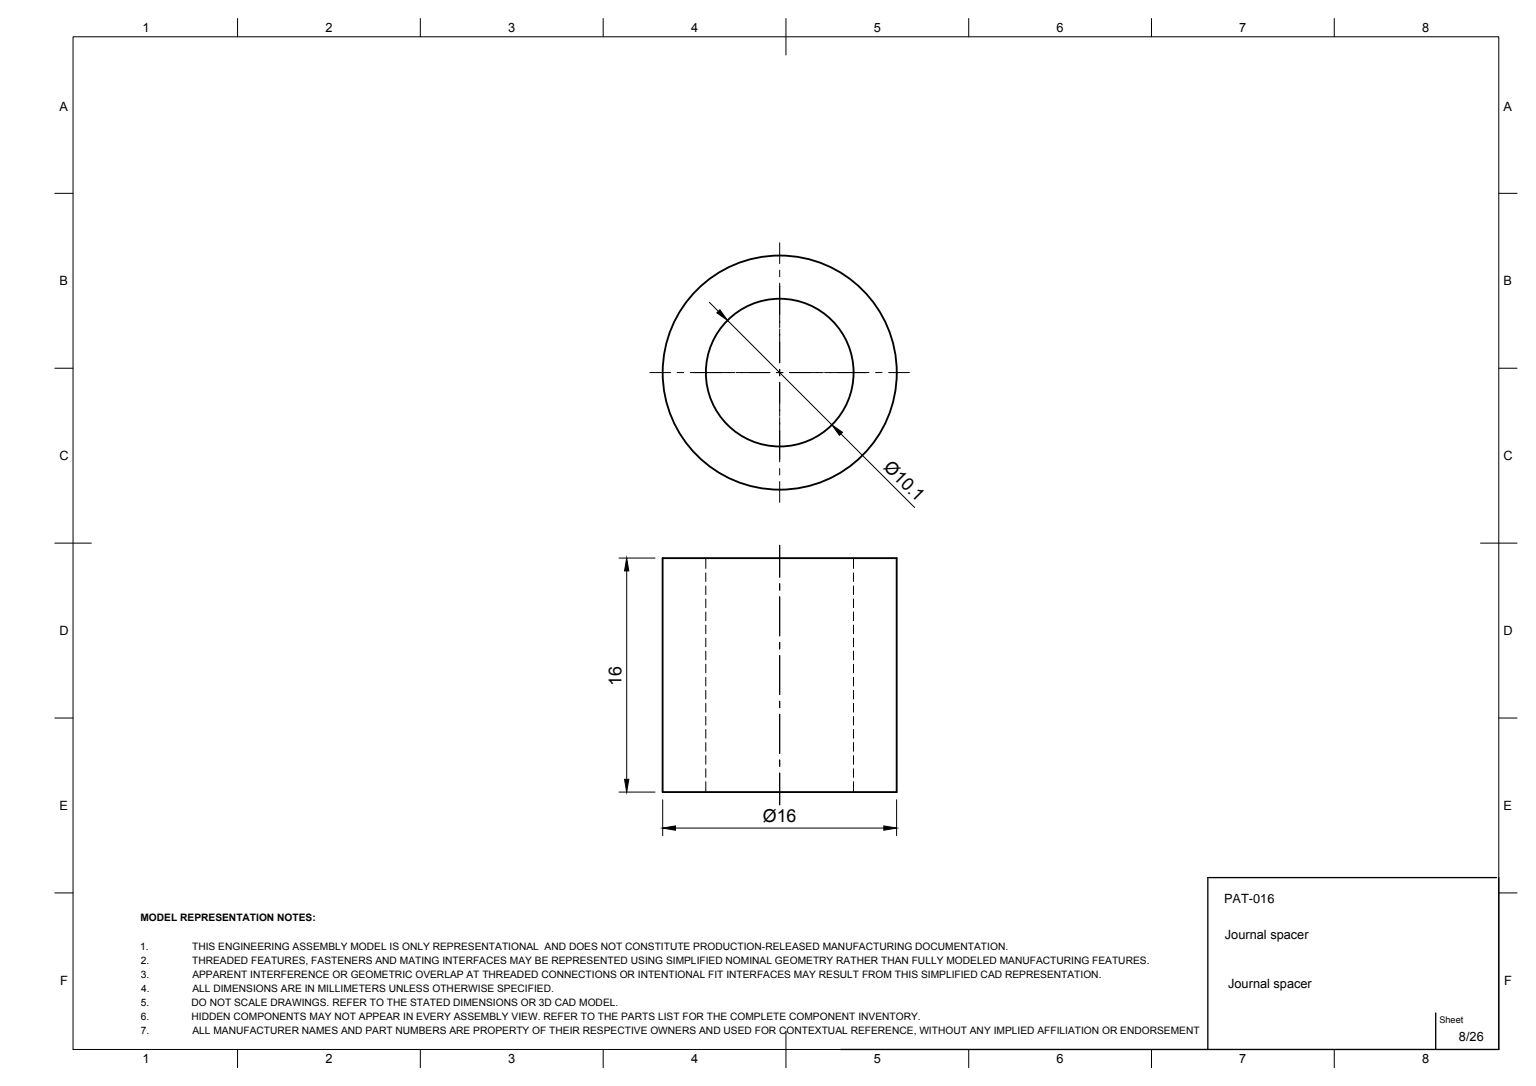
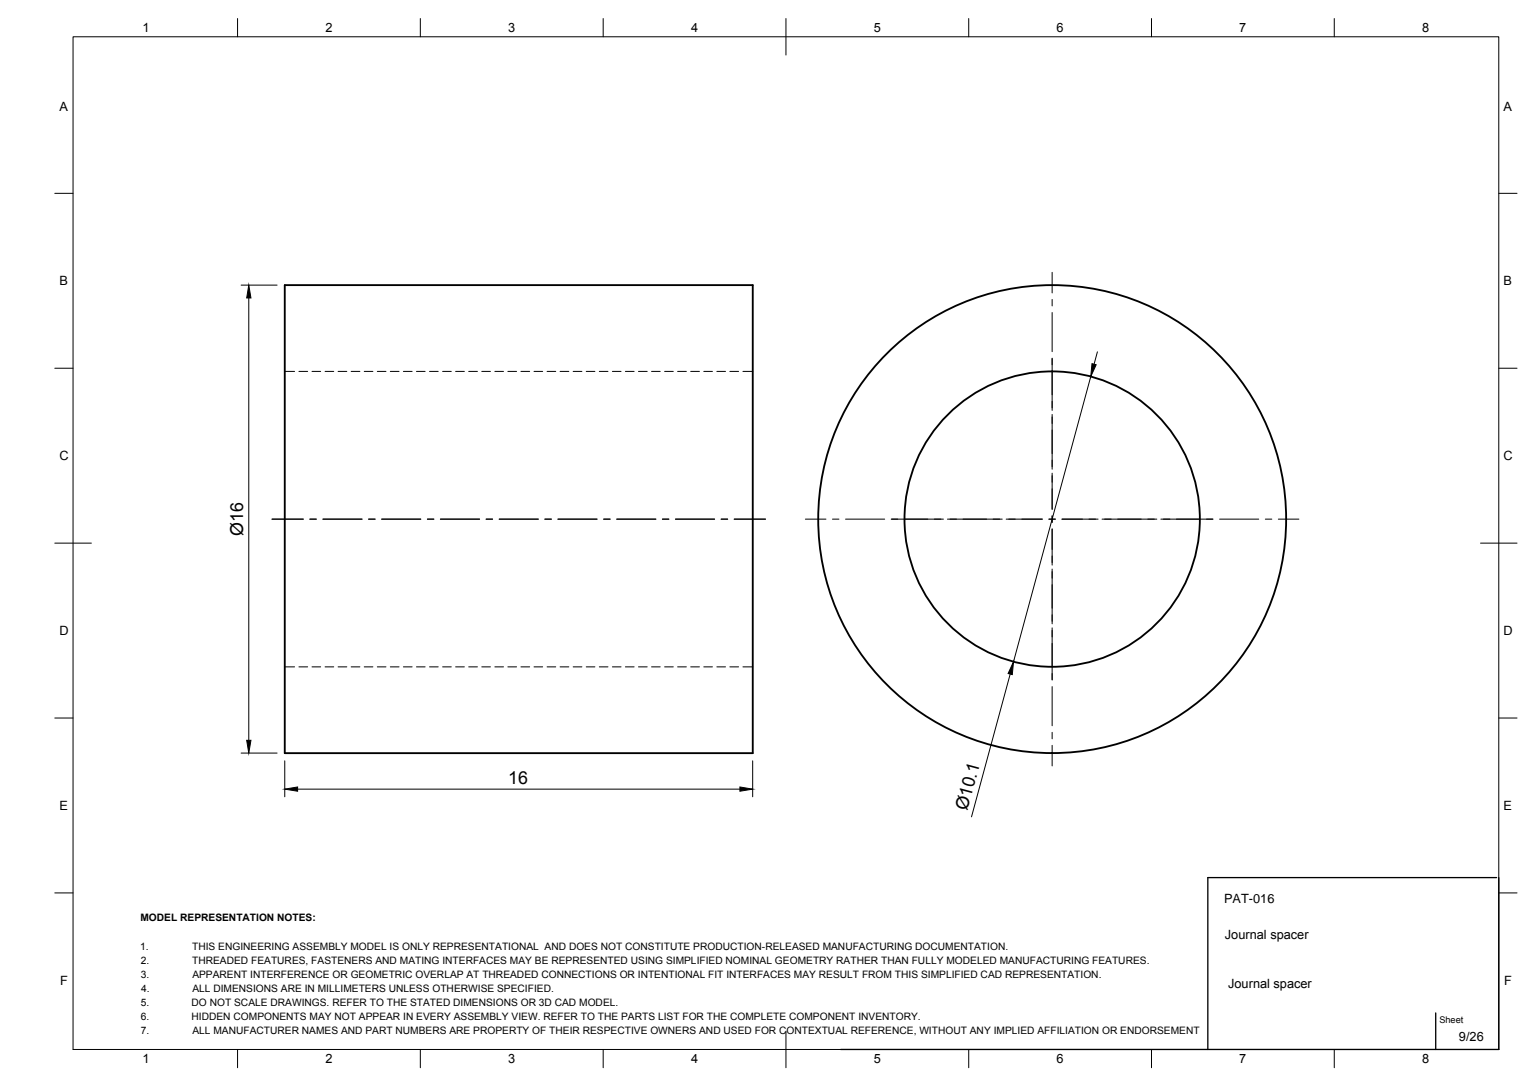
ISO-10303-21;
HEADER;
/* Generated by software containing ST-Developer
 * from STEP Tools, Inc. (www.steptools.com) 
 */

FILE_DESCRIPTION(
/* description */ ('Bracket-mounted idler roller'),
/* implementation_level */ '2;1');

FILE_NAME(
/* name */ 'Journal spacer.step',
/* time_stamp */ '2026-10-28T03:26:42-07:00',
/* author */ (''),
/* organization */ (''),
/* preprocessor_version */ 'ST-DEVELOPER v20.2',
/* originating_system */ 'Autodesk Translation Framework v15.17.0.0',
/* authorisation */ '');

FILE_SCHEMA (('AUTOMOTIVE_DESIGN { 1 0 10303 214 3 1 1 }'));
ENDSEC;

DATA;
#10=MECHANICAL_DESIGN_GEOMETRIC_PRESENTATION_REPRESENTATION('',(#283),#6241);
#241=SHAPE_REPRESENTATION_RELATIONSHIP('SRR','None',#6345,#262);
#262=ADVANCED_BREP_SHAPE_REPRESENTATION('',(#312),#6221);
#283=STYLED_ITEM('',(#6531),#312);
#312=MANIFOLD_SOLID_BREP('Body1',#3185);
#354=FACE_BOUND('',#767,.T.);
#355=FACE_BOUND('',#769,.T.);
#445=PLANE('',#3518);
#446=PLANE('',#3519);
#555=FACE_OUTER_BOUND('',#764,.T.);
#556=FACE_OUTER_BOUND('',#765,.T.);
#557=FACE_OUTER_BOUND('',#766,.T.);
#558=FACE_OUTER_BOUND('',#768,.T.);
#764=EDGE_LOOP('',(#2328,#2329,#2330,#2331));
#765=EDGE_LOOP('',(#2332,#2333,#2334,#2335));
#766=EDGE_LOOP('',(#2336));
#767=EDGE_LOOP('',(#2337));
#768=EDGE_LOOP('',(#2338));
#769=EDGE_LOOP('',(#2339));
#1038=LINE('',#5134,#1220);
#1039=LINE('',#5140,#1221);
#1220=VECTOR('',#4083,0.505);
#1221=VECTOR('',#4090,0.8);
#1365=CIRCLE('',#3513,0.505);
#1366=CIRCLE('',#3514,0.505);
#1367=CIRCLE('',#3516,0.8);
#1368=CIRCLE('',#3517,0.8);
#1578=VERTEX_POINT('',#5131);
#1579=VERTEX_POINT('',#5133);
#1580=VERTEX_POINT('',#5137);
#1581=VERTEX_POINT('',#5139);
#1866=EDGE_CURVE('',#1578,#1578,#1365,.T.);
#1867=EDGE_CURVE('',#1578,#1579,#1038,.T.);
#1868=EDGE_CURVE('',#1579,#1579,#1366,.T.);
#1869=EDGE_CURVE('',#1580,#1580,#1367,.T.);
#1870=EDGE_CURVE('',#1580,#1581,#1039,.T.);
#1871=EDGE_CURVE('',#1581,#1581,#1368,.T.);
#2328=ORIENTED_EDGE('',*,*,#1866,.F.);
#2329=ORIENTED_EDGE('',*,*,#1867,.T.);
#2330=ORIENTED_EDGE('',*,*,#1868,.T.);
#2331=ORIENTED_EDGE('',*,*,#1867,.F.);
#2332=ORIENTED_EDGE('',*,*,#1869,.F.);
#2333=ORIENTED_EDGE('',*,*,#1870,.T.);
#2334=ORIENTED_EDGE('',*,*,#1871,.T.);
#2335=ORIENTED_EDGE('',*,*,#1870,.F.);
#2336=ORIENTED_EDGE('',*,*,#1869,.T.);
#2337=ORIENTED_EDGE('',*,*,#1866,.T.);
#2338=ORIENTED_EDGE('',*,*,#1871,.F.);
#2339=ORIENTED_EDGE('',*,*,#1868,.F.);
#2939=CYLINDRICAL_SURFACE('',#3512,0.505);
#2940=CYLINDRICAL_SURFACE('',#3515,0.8);
#3030=ADVANCED_FACE('',(#555),#2939,.F.);
#3031=ADVANCED_FACE('',(#556),#2940,.T.);
#3032=ADVANCED_FACE('',(#557,#354),#445,.T.);
#3033=ADVANCED_FACE('',(#558,#355),#446,.F.);
#3185=CLOSED_SHELL('',(#3030,#3031,#3032,#3033));
#3511=AXIS2_PLACEMENT_3D('',#5129,#4077,#4078);
#3512=AXIS2_PLACEMENT_3D('',#5130,#4079,#4080);
#3513=AXIS2_PLACEMENT_3D('',#5132,#4081,#4082);
#3514=AXIS2_PLACEMENT_3D('',#5135,#4084,#4085);
#3515=AXIS2_PLACEMENT_3D('',#5136,#4086,#4087);
#3516=AXIS2_PLACEMENT_3D('',#5138,#4088,#4089);
#3517=AXIS2_PLACEMENT_3D('',#5141,#4091,#4092);
#3518=AXIS2_PLACEMENT_3D('',#5142,#4093,#4094);
#3519=AXIS2_PLACEMENT_3D('',#5143,#4095,#4096);
#4077=DIRECTION('axis',(0.,0.,1.));
#4078=DIRECTION('refdir',(1.,0.,0.));
#4079=DIRECTION('center_axis',(0.,1.,0.));
#4080=DIRECTION('ref_axis',(1.,0.,0.));
#4081=DIRECTION('center_axis',(0.,-1.,0.));
#4082=DIRECTION('ref_axis',(1.,0.,0.));
#4083=DIRECTION('',(0.,-1.,0.));
#4084=DIRECTION('center_axis',(0.,-1.,0.));
#4085=DIRECTION('ref_axis',(1.,0.,0.));
#4086=DIRECTION('center_axis',(0.,1.,0.));
#4087=DIRECTION('ref_axis',(1.,0.,0.));
#4088=DIRECTION('center_axis',(0.,1.,0.));
#4089=DIRECTION('ref_axis',(1.,0.,0.));
#4090=DIRECTION('',(0.,-1.,0.));
#4091=DIRECTION('center_axis',(0.,1.,0.));
#4092=DIRECTION('ref_axis',(1.,0.,0.));
#4093=DIRECTION('center_axis',(0.,1.,0.));
#4094=DIRECTION('ref_axis',(1.,0.,0.));
#4095=DIRECTION('center_axis',(0.,1.,0.));
#4096=DIRECTION('ref_axis',(1.,0.,0.));
#5129=CARTESIAN_POINT('',(0.,0.,0.));
#5130=CARTESIAN_POINT('Origin',(0.,-1.6,4.5));
#5131=CARTESIAN_POINT('',(-0.505,0.,4.5));
#5132=CARTESIAN_POINT('Origin',(0.,0.,4.5));
#5133=CARTESIAN_POINT('',(-0.505,-1.6,4.5));
#5134=CARTESIAN_POINT('',(-0.505,-1.6,4.5));
#5135=CARTESIAN_POINT('Origin',(0.,-1.6,4.5));
#5136=CARTESIAN_POINT('Origin',(0.,-1.6,4.5));
#5137=CARTESIAN_POINT('',(-0.8,0.,4.5));
#5138=CARTESIAN_POINT('Origin',(0.,0.,4.5));
#5139=CARTESIAN_POINT('',(-0.8,-1.6,4.5));
#5140=CARTESIAN_POINT('',(-0.8,-1.6,4.5));
#5141=CARTESIAN_POINT('Origin',(0.,-1.6,4.5));
#5142=CARTESIAN_POINT('Origin',(0.,0.,4.5));
#5143=CARTESIAN_POINT('Origin',(0.,-1.6,4.5));
#6195=UNCERTAINTY_MEASURE_WITH_UNIT(LENGTH_MEASURE(0.001),#6242,
'DISTANCE_ACCURACY_VALUE',
'Maximum model space distance between geometric entities at asserted c
onnectivities');
#6215=UNCERTAINTY_MEASURE_WITH_UNIT(LENGTH_MEASURE(0.001),#6242,
'DISTANCE_ACCURACY_VALUE',
'Maximum model space distance between geometric entities at asserted c
onnectivities');
#6221=(
GEOMETRIC_REPRESENTATION_CONTEXT(3)
GLOBAL_UNCERTAINTY_ASSIGNED_CONTEXT((#6195))
GLOBAL_UNIT_ASSIGNED_CONTEXT((#6242,#6244,#6245))
REPRESENTATION_CONTEXT('','3D')
);
#6241=(
GEOMETRIC_REPRESENTATION_CONTEXT(3)
GLOBAL_UNCERTAINTY_ASSIGNED_CONTEXT((#6215))
GLOBAL_UNIT_ASSIGNED_CONTEXT((#6242,#6244,#6245))
REPRESENTATION_CONTEXT('','3D')
);
#6242=(
LENGTH_UNIT()
NAMED_UNIT(*)
SI_UNIT(.CENTI.,.METRE.)
);
#6244=(
NAMED_UNIT(*)
PLANE_ANGLE_UNIT()
SI_UNIT($,.RADIAN.)
);
#6245=(
NAMED_UNIT(*)
SI_UNIT($,.STERADIAN.)
SOLID_ANGLE_UNIT()
);
#6251=SHAPE_DEFINITION_REPRESENTATION(#6276,#6345);
#6276=PRODUCT_DEFINITION_SHAPE('',$,#6371);
#6345=SHAPE_REPRESENTATION('',(#3511),#6221);
#6365=PRODUCT_DEFINITION_CONTEXT('part definition',#6442,'design');
#6371=PRODUCT_DEFINITION('Journal spacer','Journal spacer',#6396,#6365);
#6396=PRODUCT_DEFINITION_FORMATION('',$,#6449);
#6442=APPLICATION_CONTEXT(
'Core Data for Automotive Mechanical Design Process');
#6443=PRODUCT_CONTEXT('part definition',#6442,'mechanical');
#6449=PRODUCT('Journal spacer','Journal spacer','Journal spacer',(#6443));
#6525=COLOUR_RGB('Sky Blue',0.24,0.69,0.87);
#6526=FILL_AREA_STYLE_COLOUR('',#6525);
#6527=FILL_AREA_STYLE('',(#6526));
#6528=SURFACE_STYLE_FILL_AREA(#6527);
#6529=SURFACE_SIDE_STYLE('',(#6528));
#6530=SURFACE_STYLE_USAGE(.BOTH.,#6529);
#6531=PRESENTATION_STYLE_ASSIGNMENT((#6530));
ENDSEC;
END-ISO-10303-21;
